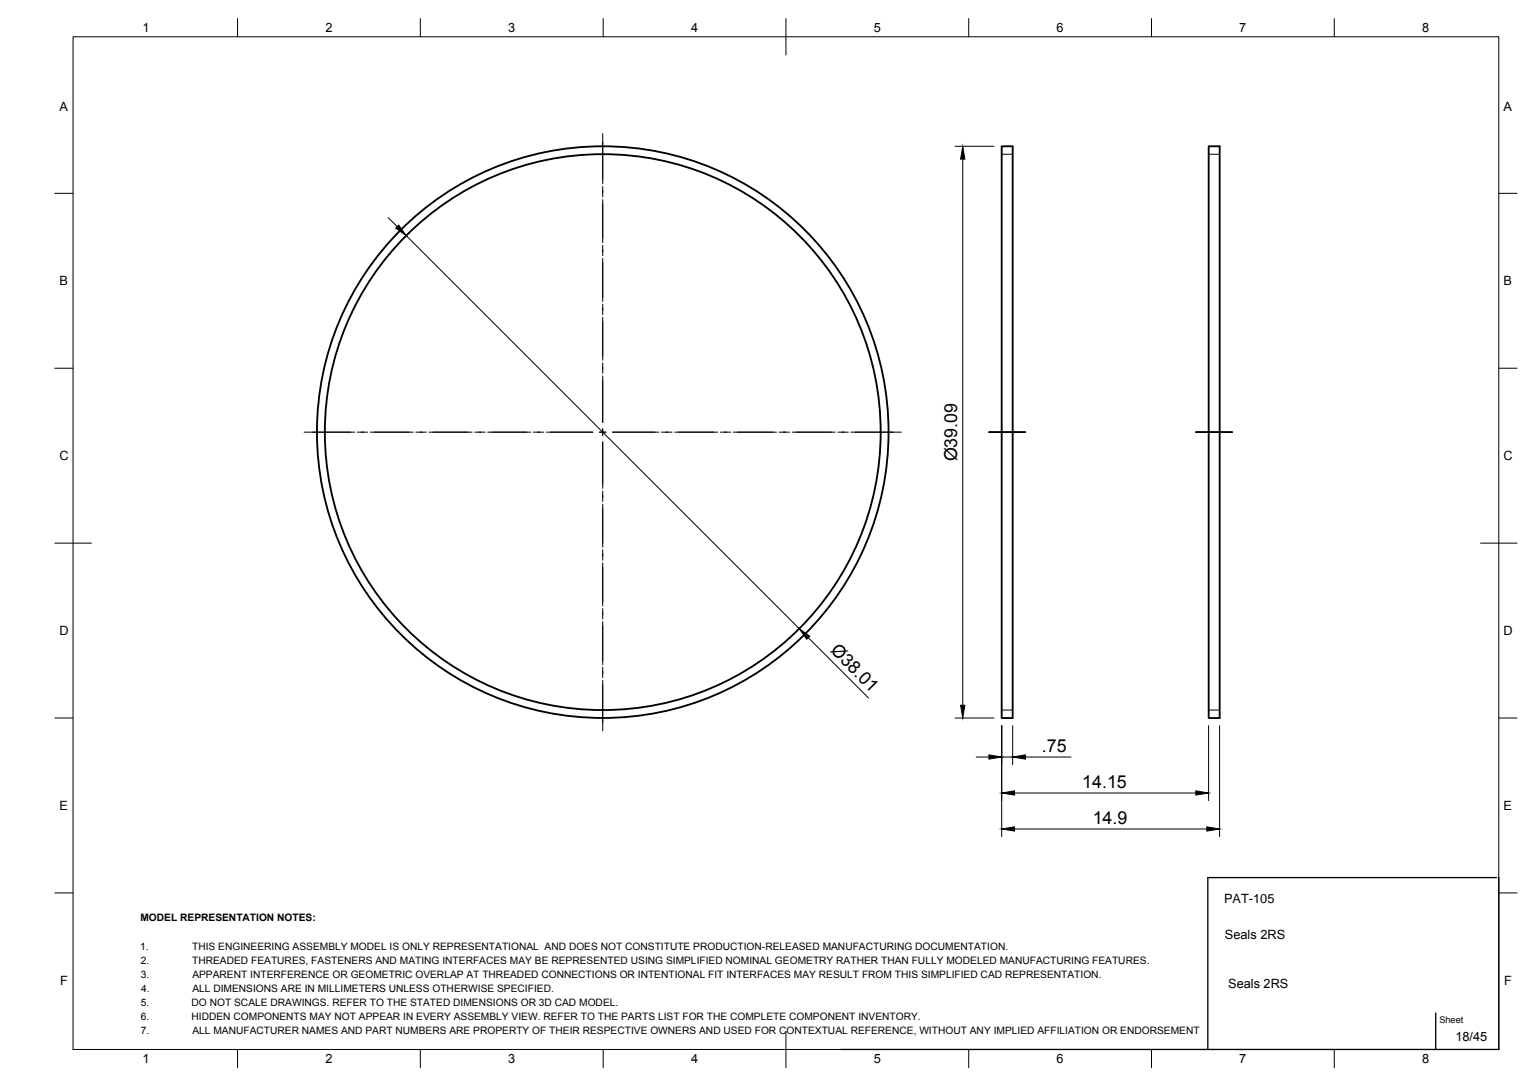
ISO-10303-21;
HEADER;
/* Generated by software containing ST-Developer
 * from STEP Tools, Inc. (www.steptools.com) 
 */

FILE_DESCRIPTION(
/* description */ ('Torque wrench calibration arm'),
/* implementation_level */ '2;1');

FILE_NAME(
/* name */ 'Seals 2RS.step',
/* time_stamp */ '2026-10-28T03:24:52-07:00',
/* author */ (''),
/* organization */ (''),
/* preprocessor_version */ 'ST-DEVELOPER v20.2',
/* originating_system */ 'Autodesk Translation Framework v15.17.0.0',
/* authorisation */ '');

FILE_SCHEMA (('AUTOMOTIVE_DESIGN { 1 0 10303 214 3 1 1 }'));
ENDSEC;

DATA;
#10=MECHANICAL_DESIGN_GEOMETRIC_PRESENTATION_REPRESENTATION('',(#445,#446),#12783);
#363=SHAPE_REPRESENTATION_RELATIONSHIP('SRR','None',#12945,#400);
#400=ADVANCED_BREP_SHAPE_REPRESENTATION('',(#499,#500),#12754);
#445=STYLED_ITEM('',(#13212),#499);
#446=STYLED_ITEM('',(#13212),#500);
#499=MANIFOLD_SOLID_BREP('Body1',#6514);
#500=MANIFOLD_SOLID_BREP('Body2',#6515);
#588=FACE_BOUND('',#1474,.T.);
#589=FACE_BOUND('',#1477,.T.);
#590=FACE_BOUND('',#1480,.T.);
#591=FACE_BOUND('',#1483,.T.);
#724=PLANE('',#7280);
#725=PLANE('',#7285);
#726=PLANE('',#7288);
#727=PLANE('',#7293);
#1021=FACE_OUTER_BOUND('',#1473,.T.);
#1022=FACE_OUTER_BOUND('',#1475,.T.);
#1023=FACE_OUTER_BOUND('',#1476,.T.);
#1024=FACE_OUTER_BOUND('',#1478,.T.);
#1025=FACE_OUTER_BOUND('',#1479,.T.);
#1026=FACE_OUTER_BOUND('',#1481,.T.);
#1027=FACE_OUTER_BOUND('',#1482,.T.);
#1028=FACE_OUTER_BOUND('',#1484,.T.);
#1473=EDGE_LOOP('',(#4997));
#1474=EDGE_LOOP('',(#4998));
#1475=EDGE_LOOP('',(#4999,#5000,#5001,#5002));
#1476=EDGE_LOOP('',(#5003));
#1477=EDGE_LOOP('',(#5004));
#1478=EDGE_LOOP('',(#5005,#5006,#5007,#5008));
#1479=EDGE_LOOP('',(#5009));
#1480=EDGE_LOOP('',(#5010));
#1481=EDGE_LOOP('',(#5011,#5012,#5013,#5014));
#1482=EDGE_LOOP('',(#5015));
#1483=EDGE_LOOP('',(#5016));
#1484=EDGE_LOOP('',(#5017,#5018,#5019,#5020));
#1932=LINE('',#11021,#2347);
#1933=LINE('',#11026,#2348);
#1934=LINE('',#11035,#2349);
#1935=LINE('',#11040,#2350);
#2347=VECTOR('',#8606,1.95469);
#2348=VECTOR('',#8613,1.90031);
#2349=VECTOR('',#8624,1.95469);
#2350=VECTOR('',#8631,1.90031);
#2775=CIRCLE('',#7281,1.95469);
#2776=CIRCLE('',#7282,1.90031);
#2777=CIRCLE('',#7284,1.95469);
#2778=CIRCLE('',#7286,1.90031);
#2779=CIRCLE('',#7289,1.95469);
#2780=CIRCLE('',#7290,1.90031);
#2781=CIRCLE('',#7292,1.95469);
#2782=CIRCLE('',#7294,1.90031);
#3197=VERTEX_POINT('',#11014);
#3198=VERTEX_POINT('',#11016);
#3199=VERTEX_POINT('',#11019);
#3200=VERTEX_POINT('',#11023);
#3201=VERTEX_POINT('',#11028);
#3202=VERTEX_POINT('',#11030);
#3203=VERTEX_POINT('',#11033);
#3204=VERTEX_POINT('',#11037);
#3856=EDGE_CURVE('',#3197,#3197,#2775,.T.);
#3857=EDGE_CURVE('',#3198,#3198,#2776,.T.);
#3858=EDGE_CURVE('',#3199,#3199,#2777,.T.);
#3859=EDGE_CURVE('',#3199,#3197,#1932,.T.);
#3860=EDGE_CURVE('',#3200,#3200,#2778,.T.);
#3861=EDGE_CURVE('',#3200,#3198,#1933,.T.);
#3862=EDGE_CURVE('',#3201,#3201,#2779,.T.);
#3863=EDGE_CURVE('',#3202,#3202,#2780,.T.);
#3864=EDGE_CURVE('',#3203,#3203,#2781,.T.);
#3865=EDGE_CURVE('',#3203,#3201,#1934,.T.);
#3866=EDGE_CURVE('',#3204,#3204,#2782,.T.);
#3867=EDGE_CURVE('',#3204,#3202,#1935,.T.);
#4997=ORIENTED_EDGE('',*,*,#3856,.F.);
#4998=ORIENTED_EDGE('',*,*,#3857,.T.);
#4999=ORIENTED_EDGE('',*,*,#3858,.F.);
#5000=ORIENTED_EDGE('',*,*,#3859,.T.);
#5001=ORIENTED_EDGE('',*,*,#3856,.T.);
#5002=ORIENTED_EDGE('',*,*,#3859,.F.);
#5003=ORIENTED_EDGE('',*,*,#3858,.T.);
#5004=ORIENTED_EDGE('',*,*,#3860,.F.);
#5005=ORIENTED_EDGE('',*,*,#3860,.T.);
#5006=ORIENTED_EDGE('',*,*,#3861,.T.);
#5007=ORIENTED_EDGE('',*,*,#3857,.F.);
#5008=ORIENTED_EDGE('',*,*,#3861,.F.);
#5009=ORIENTED_EDGE('',*,*,#3862,.F.);
#5010=ORIENTED_EDGE('',*,*,#3863,.T.);
#5011=ORIENTED_EDGE('',*,*,#3864,.F.);
#5012=ORIENTED_EDGE('',*,*,#3865,.T.);
#5013=ORIENTED_EDGE('',*,*,#3862,.T.);
#5014=ORIENTED_EDGE('',*,*,#3865,.F.);
#5015=ORIENTED_EDGE('',*,*,#3864,.T.);
#5016=ORIENTED_EDGE('',*,*,#3866,.F.);
#5017=ORIENTED_EDGE('',*,*,#3866,.T.);
#5018=ORIENTED_EDGE('',*,*,#3867,.T.);
#5019=ORIENTED_EDGE('',*,*,#3863,.F.);
#5020=ORIENTED_EDGE('',*,*,#3867,.F.);
#6037=CYLINDRICAL_SURFACE('',#7283,1.95469);
#6038=CYLINDRICAL_SURFACE('',#7287,1.90031);
#6039=CYLINDRICAL_SURFACE('',#7291,1.95469);
#6040=CYLINDRICAL_SURFACE('',#7295,1.90031);
#6246=ADVANCED_FACE('',(#1021,#588),#724,.T.);
#6247=ADVANCED_FACE('',(#1022),#6037,.T.);
#6248=ADVANCED_FACE('',(#1023,#589),#725,.T.);
#6249=ADVANCED_FACE('',(#1024),#6038,.F.);
#6250=ADVANCED_FACE('',(#1025,#590),#726,.T.);
#6251=ADVANCED_FACE('',(#1026),#6039,.T.);
#6252=ADVANCED_FACE('',(#1027,#591),#727,.T.);
#6253=ADVANCED_FACE('',(#1028),#6040,.F.);
#6514=CLOSED_SHELL('',(#6246,#6247,#6248,#6249));
#6515=CLOSED_SHELL('',(#6250,#6251,#6252,#6253));
#7279=AXIS2_PLACEMENT_3D('',#11012,#8594,#8595);
#7280=AXIS2_PLACEMENT_3D('',#11013,#8596,#8597);
#7281=AXIS2_PLACEMENT_3D('',#11015,#8598,#8599);
#7282=AXIS2_PLACEMENT_3D('',#11017,#8600,#8601);
#7283=AXIS2_PLACEMENT_3D('',#11018,#8602,#8603);
#7284=AXIS2_PLACEMENT_3D('',#11020,#8604,#8605);
#7285=AXIS2_PLACEMENT_3D('',#11022,#8607,#8608);
#7286=AXIS2_PLACEMENT_3D('',#11024,#8609,#8610);
#7287=AXIS2_PLACEMENT_3D('',#11025,#8611,#8612);
#7288=AXIS2_PLACEMENT_3D('',#11027,#8614,#8615);
#7289=AXIS2_PLACEMENT_3D('',#11029,#8616,#8617);
#7290=AXIS2_PLACEMENT_3D('',#11031,#8618,#8619);
#7291=AXIS2_PLACEMENT_3D('',#11032,#8620,#8621);
#7292=AXIS2_PLACEMENT_3D('',#11034,#8622,#8623);
#7293=AXIS2_PLACEMENT_3D('',#11036,#8625,#8626);
#7294=AXIS2_PLACEMENT_3D('',#11038,#8627,#8628);
#7295=AXIS2_PLACEMENT_3D('',#11039,#8629,#8630);
#8594=DIRECTION('axis',(0.,0.,1.));
#8595=DIRECTION('refdir',(1.,0.,0.));
#8596=DIRECTION('center_axis',(0.,1.,0.));
#8597=DIRECTION('ref_axis',(0.,0.,1.));
#8598=DIRECTION('center_axis',(0.,-1.,0.));
#8599=DIRECTION('ref_axis',(1.,0.,0.));
#8600=DIRECTION('center_axis',(0.,-1.,0.));
#8601=DIRECTION('ref_axis',(1.,0.,0.));
#8602=DIRECTION('center_axis',(0.,-1.,0.));
#8603=DIRECTION('ref_axis',(1.,0.,0.));
#8604=DIRECTION('center_axis',(0.,-1.,0.));
#8605=DIRECTION('ref_axis',(1.,0.,0.));
#8606=DIRECTION('',(0.,1.,0.));
#8607=DIRECTION('center_axis',(0.,-1.,0.));
#8608=DIRECTION('ref_axis',(0.,0.,-1.));
#8609=DIRECTION('center_axis',(0.,-1.,0.));
#8610=DIRECTION('ref_axis',(1.,0.,0.));
#8611=DIRECTION('center_axis',(0.,-1.,0.));
#8612=DIRECTION('ref_axis',(1.,0.,0.));
#8613=DIRECTION('',(0.,1.,0.));
#8614=DIRECTION('center_axis',(0.,1.,0.));
#8615=DIRECTION('ref_axis',(0.,0.,1.));
#8616=DIRECTION('center_axis',(0.,-1.,0.));
#8617=DIRECTION('ref_axis',(1.,0.,0.));
#8618=DIRECTION('center_axis',(0.,-1.,0.));
#8619=DIRECTION('ref_axis',(1.,0.,0.));
#8620=DIRECTION('center_axis',(0.,-1.,0.));
#8621=DIRECTION('ref_axis',(1.,0.,0.));
#8622=DIRECTION('center_axis',(0.,-1.,0.));
#8623=DIRECTION('ref_axis',(1.,0.,0.));
#8624=DIRECTION('',(0.,1.,0.));
#8625=DIRECTION('center_axis',(0.,-1.,0.));
#8626=DIRECTION('ref_axis',(0.,0.,-1.));
#8627=DIRECTION('center_axis',(0.,-1.,0.));
#8628=DIRECTION('ref_axis',(1.,0.,0.));
#8629=DIRECTION('center_axis',(0.,-1.,0.));
#8630=DIRECTION('ref_axis',(1.,0.,0.));
#8631=DIRECTION('',(0.,1.,0.));
#11012=CARTESIAN_POINT('',(0.,0.,0.));
#11013=CARTESIAN_POINT('Origin',(1.95469,0.745,0.));
#11014=CARTESIAN_POINT('',(-1.95469,0.745,-2.39380485182534E-16));
#11015=CARTESIAN_POINT('Origin',(0.,0.745,0.));
#11016=CARTESIAN_POINT('',(-1.90031,0.745,-2.32720855888771E-16));
#11017=CARTESIAN_POINT('Origin',(0.,0.745,0.));
#11018=CARTESIAN_POINT('Origin',(0.,0.7075,0.));
#11019=CARTESIAN_POINT('',(-1.95469,0.67,-2.39380485182534E-16));
#11020=CARTESIAN_POINT('Origin',(0.,0.67,0.));
#11021=CARTESIAN_POINT('',(-1.95469,0.7075,-2.39380485182534E-16));
#11022=CARTESIAN_POINT('Origin',(1.90031,0.67,0.));
#11023=CARTESIAN_POINT('',(-1.90031,0.67,-2.32720855888771E-16));
#11024=CARTESIAN_POINT('Origin',(0.,0.67,0.));
#11025=CARTESIAN_POINT('Origin',(0.,0.7075,0.));
#11026=CARTESIAN_POINT('',(-1.90031,0.7075,-2.32720855888771E-16));
#11027=CARTESIAN_POINT('Origin',(1.95469,-0.67,0.));
#11028=CARTESIAN_POINT('',(-1.95469,-0.67,-2.39380485182534E-16));
#11029=CARTESIAN_POINT('Origin',(0.,-0.67,0.));
#11030=CARTESIAN_POINT('',(-1.90031,-0.67,-2.32720855888771E-16));
#11031=CARTESIAN_POINT('Origin',(0.,-0.67,0.));
#11032=CARTESIAN_POINT('Origin',(0.,-0.7075,0.));
#11033=CARTESIAN_POINT('',(-1.95469,-0.745,-2.39380485182534E-16));
#11034=CARTESIAN_POINT('Origin',(0.,-0.745,0.));
#11035=CARTESIAN_POINT('',(-1.95469,-0.7075,-2.39380485182534E-16));
#11036=CARTESIAN_POINT('Origin',(1.90031,-0.745,0.));
#11037=CARTESIAN_POINT('',(-1.90031,-0.745,-2.32720855888771E-16));
#11038=CARTESIAN_POINT('Origin',(0.,-0.745,0.));
#11039=CARTESIAN_POINT('Origin',(0.,-0.7075,0.));
#11040=CARTESIAN_POINT('',(-1.90031,-0.7075,-2.32720855888771E-16));
#12710=UNCERTAINTY_MEASURE_WITH_UNIT(LENGTH_MEASURE(0.001),#12784,
'DISTANCE_ACCURACY_VALUE',
'Maximum model space distance between geometric entities at asserted c
onnectivities');
#12739=UNCERTAINTY_MEASURE_WITH_UNIT(LENGTH_MEASURE(0.001),#12784,
'DISTANCE_ACCURACY_VALUE',
'Maximum model space distance between geometric entities at asserted c
onnectivities');
#12754=(
GEOMETRIC_REPRESENTATION_CONTEXT(3)
GLOBAL_UNCERTAINTY_ASSIGNED_CONTEXT((#12710))
GLOBAL_UNIT_ASSIGNED_CONTEXT((#12784,#12786,#12787))
REPRESENTATION_CONTEXT('','3D')
);
#12783=(
GEOMETRIC_REPRESENTATION_CONTEXT(3)
GLOBAL_UNCERTAINTY_ASSIGNED_CONTEXT((#12739))
GLOBAL_UNIT_ASSIGNED_CONTEXT((#12784,#12786,#12787))
REPRESENTATION_CONTEXT('','3D')
);
#12784=(
LENGTH_UNIT()
NAMED_UNIT(*)
SI_UNIT(.CENTI.,.METRE.)
);
#12786=(
NAMED_UNIT(*)
PLANE_ANGLE_UNIT()
SI_UNIT($,.RADIAN.)
);
#12787=(
NAMED_UNIT(*)
SI_UNIT($,.STERADIAN.)
SOLID_ANGLE_UNIT()
);
#12802=SHAPE_DEFINITION_REPRESENTATION(#12845,#12945);
#12845=PRODUCT_DEFINITION_SHAPE('',$,#12989);
#12945=SHAPE_REPRESENTATION('',(#7279),#12754);
#12974=PRODUCT_DEFINITION_CONTEXT('part definition',#13105,'design');
#12989=PRODUCT_DEFINITION('Seals 2RS','Seals 2RS',#13032,#12974);
#13032=PRODUCT_DEFINITION_FORMATION('',$,#13121);
#13105=APPLICATION_CONTEXT(
'Core Data for Automotive Mechanical Design Process');
#13106=PRODUCT_CONTEXT('part definition',#13105,'mechanical');
#13121=PRODUCT('Seals 2RS','Seals 2RS','Seals 2RS',(#13106));
#13206=COLOUR_RGB('Grey',0.48,0.52,0.57);
#13207=FILL_AREA_STYLE_COLOUR('',#13206);
#13208=FILL_AREA_STYLE('',(#13207));
#13209=SURFACE_STYLE_FILL_AREA(#13208);
#13210=SURFACE_SIDE_STYLE('',(#13209));
#13211=SURFACE_STYLE_USAGE(.BOTH.,#13210);
#13212=PRESENTATION_STYLE_ASSIGNMENT((#13211));
ENDSEC;
END-ISO-10303-21;
